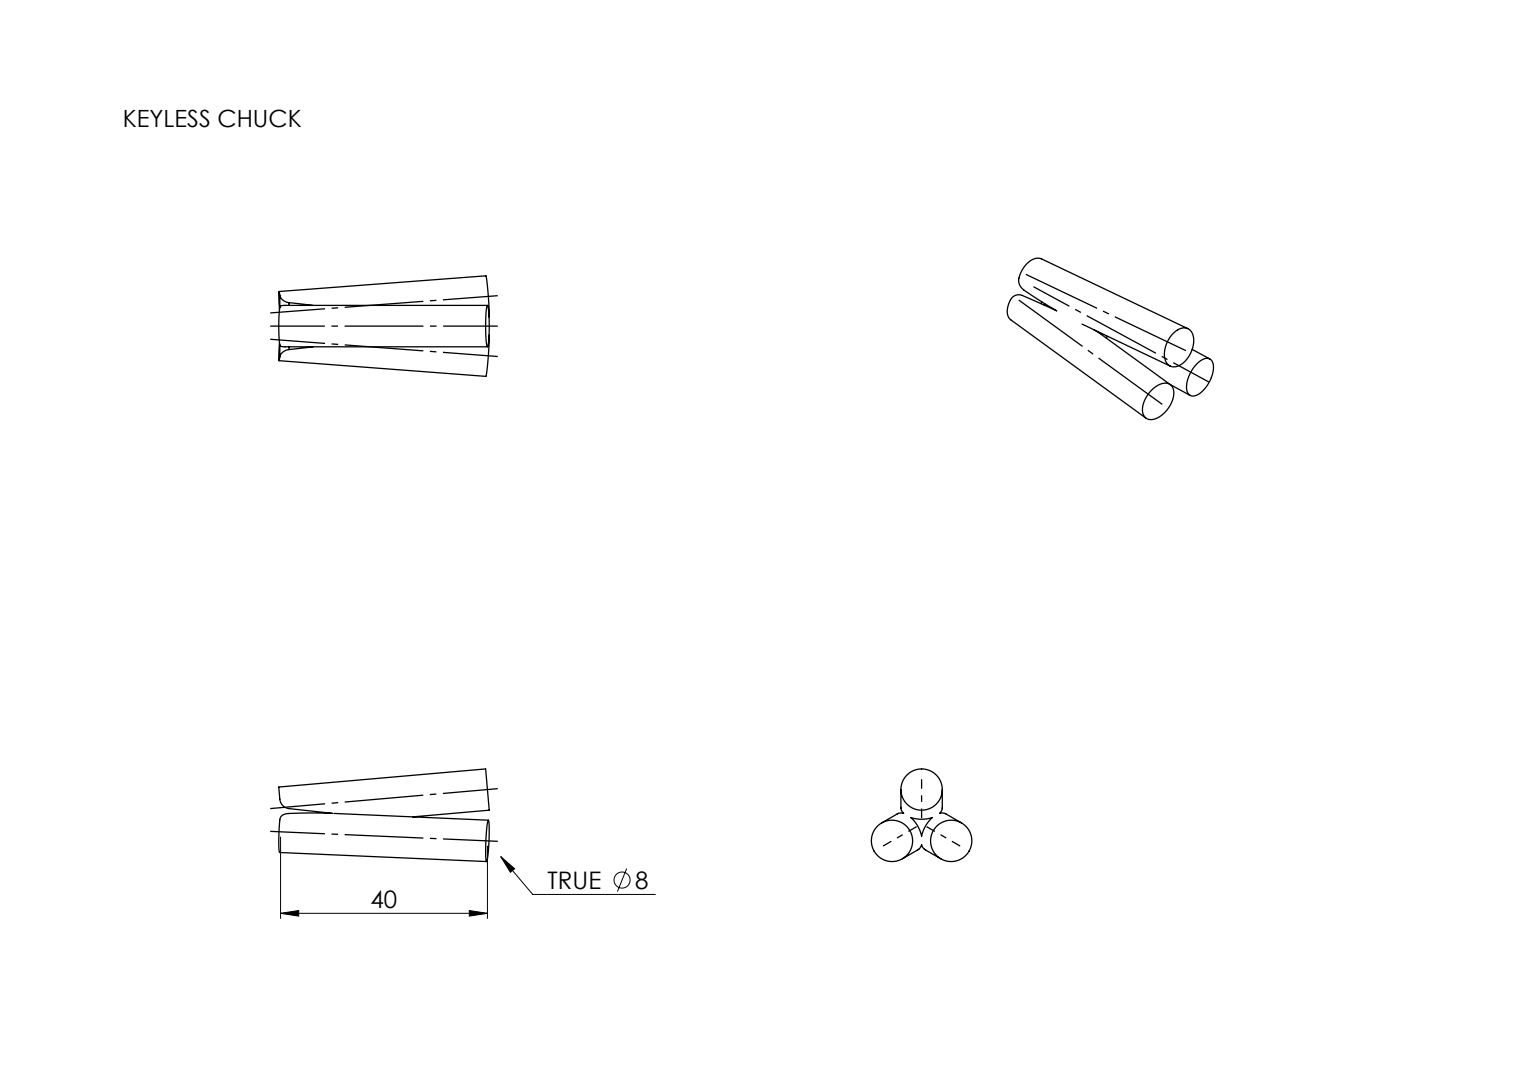
ISO-10303-21;
HEADER;
FILE_DESCRIPTION (('STEP AP214'),
    '1' );
FILE_NAME ('Keyless Chuck.step',
    '2026-10-05T20:22:16',
    ( '' ),
    ( '' ),
    'SwSTEP 2.0',
    'SolidWorks 2026',
    '' );
FILE_SCHEMA (( 'AUTOMOTIVE_DESIGN' ));
ENDSEC;

DATA;
#15=AXIS2_PLACEMENT_3D ( 'NONE', #2563, #7954, #5300 ) ;
#46=SHAPE_DEFINITION_REPRESENTATION ( #2904, #690 ) ;
#51=AXIS2_PLACEMENT_3D ( 'NONE', #14892, #2772, #6847 ) ;
#157=STYLED_ITEM ( 'NONE', ( #14231 ), #11475 ) ;
#195=DIRECTION ( 'NONE',  ( 0.1091791256177803149, 0.9940220915700701543, 0.000000000000000000 ) ) ;
#229=CARTESIAN_POINT ( 'NONE',  ( -208.1430079281944074, 172.4097984991905150, 5.932774073184737595 ) ) ;
#323=ORIENTED_EDGE ( 'NONE', *, *, #15869, .T. ) ;
#367=CARTESIAN_POINT ( 'NONE',  ( -206.3689767832464668, 174.5534660175772785, 3.987129972734268168 ) ) ;
#396=CARTESIAN_POINT ( 'NONE',  ( -206.1506185320109239, 176.5415102007174255, 53.79077198841061147 ) ) ;
#448=CARTESIAN_POINT ( 'NONE',  ( -207.5170152892447959, 175.0764231502095072, 3.989746324742934558 ) ) ;
#456=AXIS2_PLACEMENT_3D ( 'NONE', #11979, #6311, #7995 ) ;
#518=CIRCLE ( 'NONE', #8724, 4.000000000000001776 ) ;
#542=CARTESIAN_POINT ( 'NONE',  ( -187.6513770290094385, 171.1853623553244006, 0.7576236986490064718 ) ) ;
#607=EDGE_CURVE ( 'NONE', #15092, #6530, #17001, .T. ) ;
#637=CARTESIAN_POINT ( 'NONE',  ( -207.6770884633517085, 166.3723159270569738, -1.150078995496658596 ) ) ;
#638=CARTESIAN_POINT ( 'NONE',  ( -207.7508999721942189, 175.3364228813296108, 3.959069933371625716 ) ) ;
#664=CARTESIAN_POINT ( 'NONE',  ( -206.3689767832464668, 174.5534660175772785, 53.79077198841061147 ) ) ;
#686=( NAMED_UNIT ( * ) SI_UNIT ( $, .STERADIAN. ) SOLID_ANGLE_UNIT ( ) );
#690=SHAPE_REPRESENTATION ( 'Keyless Chuck', ( #3583 ), #12675 ) ;
#739=CARTESIAN_POINT ( 'NONE',  ( -195.2299705378136991, 173.3300053194287784, 3.811055608065186728 ) ) ;
#766=CARTESIAN_POINT ( 'NONE',  ( -207.6513770290094669, 172.0602489905835739, -0.7577244044828647107 ) ) ;
#773=AXIS2_PLACEMENT_3D ( 'NONE', #13462, #4256, #5749 ) ;
#777=( LENGTH_UNIT ( ) NAMED_UNIT ( * ) SI_UNIT ( .MILLI., .METRE. ) );
#789=DIRECTION ( 'NONE',  ( 0.9961946980917461003, 0.08715574274765185148, 0.000000000000000000 ) ) ;
#824=CIRCLE ( 'NONE', #2229, 3.999999999999985789 ) ;
#840=ORIENTED_EDGE ( 'NONE', *, *, #4013, .T. ) ;
#841=CARTESIAN_POINT ( 'NONE',  ( -207.2467692809710229, 174.8522807748693708, -4.001497440111938531 ) ) ;
#849=EDGE_CURVE ( 'NONE', #13616, #7959, #8196, .T. ) ;
#859=DIRECTION ( 'NONE',  ( -0.08715574274764689711, 0.9961946980917465444, 0.000000000000000000 ) ) ;
#924=ORIENTED_EDGE ( 'NONE', *, *, #4888, .T. ) ;
#935=EDGE_CURVE ( 'NONE', #15663, #15092, #15839, .T. ) ;
#944=FACE_OUTER_BOUND ( 'NONE', #7191, .T. ) ;
#1009=ORIENTED_EDGE ( 'NONE', *, *, #607, .T. ) ;
#1035=FACE_OUTER_BOUND ( 'NONE', #10686, .T. ) ;
#1091=DIRECTION ( 'NONE',  ( 0.000000000000000000, 0.8660254037844363761, 0.5000000000000039968 ) ) ;
#1110=SURFACE_STYLE_FILL_AREA ( #5093 ) ;
#1139=CARTESIAN_POINT ( 'NONE',  ( -206.6025269363104258, 173.6007587957575993, -4.555677747302790515 ) ) ;
#1184=FACE_OUTER_BOUND ( 'NONE', #5191, .T. ) ;
#1208=ORIENTED_EDGE ( 'NONE', *, *, #14941, .T. ) ;
#1212=PRESENTATION_STYLE_ASSIGNMENT (( #2453 ) ) ;
#1213=DIRECTION ( 'NONE',  ( -0.08715574274765344742, -0.4980973490458779906, 0.8627299156628184251 ) ) ;
#1262=CARTESIAN_POINT ( 'NONE',  ( -208.1430079281944074, 176.3671987152221448, 3.647967993167786194 ) ) ;
#1265=ORIENTED_EDGE ( 'NONE', *, *, #4152, .T. ) ;
#1297=STYLED_ITEM ( 'NONE', ( #15804 ), #5484 ) ;
#1302=CYLINDRICAL_SURFACE ( 'NONE', #11228, 3.999999999999999556 ) ;
#1304=CARTESIAN_POINT ( 'NONE',  ( -208.0000000000000853, 170.0678595944000620, 2.693195258168412654 ) ) ;
#1332=APPLICATION_CONTEXT ( 'automotive_design' ) ;
#1368=AXIS2_PLACEMENT_3D ( 'NONE', #14284, #2415, #6495 ) ;
#1393=AXIS2_PLACEMENT_3D ( 'NONE', #396, #7302, #5984 ) ;
#1460=VERTEX_POINT ( 'NONE', #542 ) ;
#1523=ORIENTED_EDGE ( 'NONE', *, *, #3971, .T. ) ;
#1571=FACE_OUTER_BOUND ( 'NONE', #7575, .T. ) ;
#1581=FACE_OUTER_BOUND ( 'NONE', #1905, .T. ) ;
#1616=DIRECTION ( 'NONE',  ( -0.9940220915700700433, 0.1091791256177803010, 0.000000000000000000 ) ) ;
#1619=EDGE_CURVE ( 'NONE', #10750, #7725, #11750, .T. ) ;
#1633=PRODUCT_DEFINITION_FORMATION_WITH_SPECIFIED_SOURCE ( 'ANY', '', #8716, .NOT_KNOWN. ) ;
#1648=CARTESIAN_POINT ( 'NONE',  ( -206.8260782938592968, 173.5737298318736350, 4.615523682683083884 ) ) ;
#1664=CARTESIAN_POINT ( 'NONE',  ( -208.1243352336975079, 166.1145920781434029, 2.051787360128269899 ) ) ;
#1670=AXIS2_PLACEMENT_3D ( 'NONE', #11861, #14612, #14871 ) ;
#1700=EDGE_LOOP ( 'NONE', ( #10050, #15247, #3822 ) ) ;
#1706=CARTESIAN_POINT ( 'NONE',  ( -207.9324504923922916, 166.2413418076914979, -1.515671747849433926 ) ) ;
#1748=CARTESIAN_POINT ( 'NONE',  ( -207.9328752093750836, 166.2410986792852725, 1.516464574996131409 ) ) ;
#1830=MECHANICAL_DESIGN_GEOMETRIC_PRESENTATION_REPRESENTATION('',(#15396),#8611);
#1858=ORIENTED_EDGE ( 'NONE', *, *, #13622, .T. ) ;
#1899=ADVANCED_FACE ( 'NONE', ( #1035 ), #13080, .T. ) ;
#1905=EDGE_LOOP ( 'NONE', ( #3437, #5081, #4944 ) ) ;
#1946=FACE_OUTER_BOUND ( 'NONE', #7383, .T. ) ;
#1962=CARTESIAN_POINT ( 'NONE',  ( -206.8291083847463767, 174.6458110457699320, 3.997382128395213563 ) ) ;
#2102=CARTESIAN_POINT ( 'NONE',  ( -206.3689767832464668, 173.6103877383153247, 4.531616471133065538 ) ) ;
#2132=EDGE_CURVE ( 'NONE', #16060, #12961, #14037, .T. ) ;
#2147=CLOSED_SHELL ( 'NONE', ( #14473, #16622, #2895, #16851, #8239, #12846 ) ) ;
#2222=ORIENTED_EDGE ( 'NONE', *, *, #14690, .T. ) ;
#2229=AXIS2_PLACEMENT_3D ( 'NONE', #2965, #8362, #5374 ) ;
#2260=( NAMED_UNIT ( * ) PLANE_ANGLE_UNIT ( ) SI_UNIT ( $, .RADIAN. ) );
#2263=DIRECTION ( 'NONE',  ( 0.9961946980917461003, -0.04357787137382628656, 0.07547908730516766918 ) ) ;
#2279=EDGE_LOOP ( 'NONE', ( #3266, #2377, #8282 ) ) ;
#2286=ORIENTED_EDGE ( 'NONE', *, *, #6993, .T. ) ;
#2301=ORIENTED_EDGE ( 'NONE', *, *, #5852, .T. ) ;
#2354=EDGE_CURVE ( 'NONE', #15563, #4664, #11297, .T. ) ;
#2357=CARTESIAN_POINT ( 'NONE',  ( -206.3689767832464668, 174.5534660175772785, -3.987129972734268168 ) ) ;
#2377=ORIENTED_EDGE ( 'NONE', *, *, #13820, .T. ) ;
#2389=CYLINDRICAL_SURFACE ( 'NONE', #1670, 2.000000000000001776 ) ;
#2415=DIRECTION ( 'NONE',  ( 0.1091791256177803288, -0.4970110457850271390, -0.8608483832226269117 ) ) ;
#2416=( GEOMETRIC_REPRESENTATION_CONTEXT ( 3 ) GLOBAL_UNCERTAINTY_ASSIGNED_CONTEXT ( ( #11805 ) ) GLOBAL_UNIT_ASSIGNED_CONTEXT ( ( #777, #6172, #686 ) ) REPRESENTATION_CONTEXT ( 'NONE', 'WORKASPACE' ) );
#2424=UNCERTAINTY_MEASURE_WITH_UNIT (LENGTH_MEASURE( 1.000000000000000082E-05 ), #9338, 'distance_accuracy_value', 'NONE');
#2453=SURFACE_STYLE_USAGE ( .BOTH. , #10588 ) ;
#2470=VERTEX_POINT ( 'NONE', #6364 ) ;
#2494=B_SPLINE_CURVE_WITH_KNOTS ( 'NONE', 3,
 ( #6445, #17249, #7857, #10785, #13268, #9183, #9275, #3786, #15833, #5124, #15917, #16195, #1139, #5029 ),
 .UNSPECIFIED., .F., .F.,
 ( 4, 2, 2, 2, 2, 2, 4 ),
 ( 0.000000000000000000, 0.0006954478661160458245, 0.001043171799174067707, 0.001390895732232089697, 0.001738619665290111688, 0.002086343598348133679, 0.002781791464464176359 ),
 .UNSPECIFIED. ) ;
#2514=CARTESIAN_POINT ( 'NONE',  ( -207.6770884633516516, 175.2440045654562368, -3.971992828049704993 ) ) ;
#2529=EDGE_CURVE ( 'NONE', #12961, #8416, #16124, .T. ) ;
#2558=AXIS2_PLACEMENT_3D ( 'NONE', #1304, #5022, #1213 ) ;
#2563=CARTESIAN_POINT ( 'NONE',  ( -208.0000000000000853, 123.4836845632602262, -24.20219073603711735 ) ) ;
#2589=FACE_OUTER_BOUND ( 'NONE', #7027, .T. ) ;
#2608=ORIENTED_EDGE ( 'NONE', *, *, #6258, .T. ) ;
#2655=DIRECTION ( 'NONE',  ( -0.08715574274764661955, -0.4980973490458647235, -0.8627299156628267518 ) ) ;
#2663=PRESENTATION_STYLE_ASSIGNMENT (( #7884 ) ) ;
#2666=DIRECTION ( 'NONE',  ( 0.9961946980917461003, -0.04357787137382628656, 0.07547908730516766918 ) ) ;
#2747=CARTESIAN_POINT ( 'NONE',  ( -208.0000000000000853, 174.7326106162513497, 0.000000000000000000 ) ) ;
#2751=CARTESIAN_POINT ( 'NONE',  ( -206.3689767832464668, 173.6103877383153531, -4.531616471133038004 ) ) ;
#2760=AXIS2_PLACEMENT_3D ( 'NONE', #15474, #12819, #3354 ) ;
#2772=DIRECTION ( 'NONE',  ( 0.9961946980917464334, 0.08715574274764831264, 0.000000000000000000 ) ) ;
#2796=AXIS2_PLACEMENT_3D ( 'NONE', #9390, #2666, #8056 ) ;
#2809=ORIENTED_EDGE ( 'NONE', *, *, #4152, .F. ) ;
#2813=CARTESIAN_POINT ( 'NONE',  ( -207.2426727481553996, 166.5388791023002852, 0.8050770646283873511 ) ) ;
#2859=ORIENTED_EDGE ( 'NONE', *, *, #17159, .T. ) ;
#2894=CARTESIAN_POINT ( 'NONE',  ( -207.7508999721942189, 166.3372983242019529, 1.236577052156976331 ) ) ;
#2895=ADVANCED_FACE ( 'NONE', ( #6536 ), #9267, .T. ) ;
#2904=PRODUCT_DEFINITION_SHAPE ( 'NONE', 'NONE',  #4806 ) ;
#2965=CARTESIAN_POINT ( 'NONE',  ( -168.0000000000000284, 178.2321571572880146, 0.000000000000000000 ) ) ;
#2994=DIRECTION ( 'NONE',  ( -0.08715574274764689711, 0.9961946980917465444, 0.000000000000000000 ) ) ;
#3095=DIRECTION ( 'NONE',  ( 0.9961946980917465444, -0.04357787137382451714, 0.07547908730516460218 ) ) ;
#3142=APPLICATION_CONTEXT ( 'automotive_design' ) ;
#3156=ORIENTED_EDGE ( 'NONE', *, *, #3757, .F. ) ;
#3173=EDGE_CURVE ( 'NONE', #1460, #13560, #8889, .T. ) ;
#3177=FACE_OUTER_BOUND ( 'NONE', #12170, .T. ) ;
#3266=ORIENTED_EDGE ( 'NONE', *, *, #3738, .F. ) ;
#3269=MECHANICAL_DESIGN_GEOMETRIC_PRESENTATION_REPRESENTATION('',(#157),#2416);
#3278=ORIENTED_EDGE ( 'NONE', *, *, #3173, .F. ) ;
#3350=SURFACE_STYLE_USAGE ( .BOTH. , #11477 ) ;
#3354=DIRECTION ( 'NONE',  ( -0.08715574274764828488, -0.4980973490458772135, 0.8627299156628193133 ) ) ;
#3371=CARTESIAN_POINT ( 'NONE',  ( -207.6513770290094669, 170.7478318238843542, 4.898587196589412829E-16 ) ) ;
#3404=LINE ( 'NONE', #12602, #7236 ) ;
#3437=ORIENTED_EDGE ( 'NONE', *, *, #13167, .F. ) ;
#3583=AXIS2_PLACEMENT_3D ( 'NONE', #5482, #6893, #8222 ) ;
#3595=CARTESIAN_POINT ( 'NONE',  ( -167.6513770290094385, 170.3104757200652273, -2.272971801780872880 ) ) ;
#3667=AXIS2_PLACEMENT_3D ( 'NONE', #8932, #14257, #10184 ) ;
#3693=ORIENTED_EDGE ( 'NONE', *, *, #16219, .F. ) ;
#3700=VECTOR ( 'NONE', #11958, 1000.000000000000000 ) ;
#3705=EDGE_CURVE ( 'NONE', #2470, #13560, #518, .T. ) ;
#3714=ORIENTED_EDGE ( 'NONE', *, *, #12478, .T. ) ;
#3738=EDGE_CURVE ( 'NONE', #12853, #7172, #10395, .T. ) ;
#3757=EDGE_CURVE ( 'NONE', #5890, #4664, #5665, .T. ) ;
#3783=DIRECTION ( 'NONE',  ( -0.08715574274764661955, -0.4980973490458647235, -0.8627299156628267518 ) ) ;
#3786=CARTESIAN_POINT ( 'NONE',  ( -207.5170152892447675, 173.3511749993040496, -4.985818809087040115 ) ) ;
#3822=ORIENTED_EDGE ( 'NONE', *, *, #1619, .F. ) ;
#3839=MECHANICAL_DESIGN_GEOMETRIC_PRESENTATION_REPRESENTATION('',(#1297),#13733);
#3886=CARTESIAN_POINT ( 'NONE',  ( -187.6513770290094669, 169.2829632032627103, 0.3407269638998700612 ) ) ;
#3911=VECTOR ( 'NONE', #12611, 1000.000000000000000 ) ;
#3914=( NAMED_UNIT ( * ) SI_UNIT ( $, .STERADIAN. ) SOLID_ANGLE_UNIT ( ) );
#3971=EDGE_CURVE ( 'NONE', #12127, #1460, #5551, .T. ) ;
#3978=AXIS2_PLACEMENT_3D ( 'NONE', #8826, #8563, #16727 ) ;
#4013=EDGE_CURVE ( 'NONE', #10750, #5523, #14167, .T. ) ;
#4023=CARTESIAN_POINT ( 'NONE',  ( -207.8780901672883488, 175.5271247293819386, 3.924367008119225453 ) ) ;
#4035=ORIENTED_EDGE ( 'NONE', *, *, #15780, .T. ) ;
#4127=CARTESIAN_POINT ( 'NONE',  ( -207.6770884633517653, 173.2520093125383198, 5.122071823546326286 ) ) ;
#4152=EDGE_CURVE ( 'NONE', #4664, #15793, #8244, .T. ) ;
#4193=ORIENTED_EDGE ( 'NONE', *, *, #8859, .F. ) ;
#4205=B_SPLINE_CURVE_WITH_KNOTS ( 'NONE', 3,
 ( #8099, #12190, #1648, #10846, #16259, #4127, #9427, #13517, #9512, #8194, #15086, #229 ),
 .UNSPECIFIED., .F., .F.,
 ( 4, 2, 2, 2, 2, 4 ),
 ( 0.000000000000000000, 0.0006954760458706750904, 0.001390952091741350181, 0.001738690114676716024, 0.002086428137612082300, 0.002781904183482815287 ),
 .UNSPECIFIED. ) ;
#4256=DIRECTION ( 'NONE',  ( 0.000000000000000000, 0.8660254037844363761, 0.5000000000000041078 ) ) ;
#4290=ORIENTED_EDGE ( 'NONE', *, *, #2132, .F. ) ;
#4328=DIRECTION ( 'NONE',  ( -0.08715574274764828488, -0.4980973490458772135, 0.8627299156628193133 ) ) ;
#4397=DIRECTION ( 'NONE',  ( -0.08715574274765354457, -0.4980973490458646125, -0.8627299156628260857 ) ) ;
#4408=CARTESIAN_POINT ( 'NONE',  ( -206.8291083847463199, 166.6494249078165808, 0.6193335608963369543 ) ) ;
#4417=( BOUNDED_CURVE ( )  B_SPLINE_CURVE ( 3, ( #9196, #6639, #739, #9379 ),
 .UNSPECIFIED., .F., .F. ) 
 B_SPLINE_CURVE_WITH_KNOTS ( ( 4, 4 ),
 ( 0.000000000000000000, 1.490556265852237994 ),
 .UNSPECIFIED. ) 
 CURVE ( )  GEOMETRIC_REPRESENTATION_ITEM ( )  RATIONAL_B_SPLINE_CURVE ( ( 1.000000000000000000, 0.8232662051119113977, 0.8232662051119113977, 1.000000000000000000 ) ) 
 REPRESENTATION_ITEM ( '' )  );
#4445=ORIENTED_EDGE ( 'NONE', *, *, #17458, .F. ) ;
#4448=CARTESIAN_POINT ( 'NONE',  ( -206.3689767832464668, 166.7044760491588704, -0.5444864983988328966 ) ) ;
#4449=DIRECTION ( 'NONE',  ( -0.08715574274765354457, -0.4980973490458646125, -0.8627299156628260857 ) ) ;
#4469=ORIENTED_EDGE ( 'NONE', *, *, #15780, .F. ) ;
#4496=CARTESIAN_POINT ( 'NONE',  ( -207.5170152892447675, 166.4407316555380589, 0.9960724843441398635 ) ) ;
#4557=ORIENTED_EDGE ( 'NONE', *, *, #13622, .F. ) ;
#4624=CARTESIAN_POINT ( 'NONE',  ( -207.4300157105866447, 174.9998640698394468, 3.994873866052218947 ) ) ;
#4635=CARTESIAN_POINT ( 'NONE',  ( -207.6513770290094669, 172.0602489905835171, 0.7577244044828906899 ) ) ;
#4664=VERTEX_POINT ( 'NONE', #11365 ) ;
#4806=PRODUCT_DEFINITION ( 'UNKNOWN', '', #1633, #16115 ) ;
#4847=DIRECTION ( 'NONE',  ( 0.9961946980917465444, -0.04357787137382451714, 0.07547908730516460218 ) ) ;
#4852=CARTESIAN_POINT ( 'NONE',  ( -187.6513770290094669, 172.4976050944027008, -2.196701325097758062 ) ) ;
#4888=EDGE_CURVE ( 'NONE', #7725, #17193, #10115, .T. ) ;
#4896=ADVANCED_FACE ( 'NONE', ( #5768 ), #15411, .T. ) ;
#4898=LINE ( 'NONE', #11887, #8985 ) ;
#4944=ORIENTED_EDGE ( 'NONE', *, *, #2354, .F. ) ;
#4975=ORIENTED_EDGE ( 'NONE', *, *, #13167, .T. ) ;
#5022=DIRECTION ( 'NONE',  ( 0.9961946980917461003, -0.04357787137382628656, 0.07547908730516766918 ) ) ;
#5029=CARTESIAN_POINT ( 'NONE',  ( -206.3689767832464668, 173.6103877383153531, -4.531616471133038004 ) ) ;
#5039=ORIENTED_EDGE ( 'NONE', *, *, #10242, .F. ) ;
#5081=ORIENTED_EDGE ( 'NONE', *, *, #3757, .T. ) ;
#5093=FILL_AREA_STYLE ('',( #5264 ) ) ;
#5124=CARTESIAN_POINT ( 'NONE',  ( -207.2426727481553996, 173.4675081614032877, -4.805322917016542128 ) ) ;
#5191=EDGE_LOOP ( 'NONE', ( #9064, #9073, #1208, #3714, #840, #4469 ) ) ;
#5264=FILL_AREA_STYLE_COLOUR ( '', #16842 ) ;
#5282=STYLED_ITEM ( 'NONE', ( #1212 ), #12908 ) ;
#5300=DIRECTION ( 'NONE',  ( -0.9940220915700700433, -0.05458956280889060153, 0.09455189634796991316 ) ) ;
#5306=AXIS2_PLACEMENT_3D ( 'NONE', #9251, #4847, #8988 ) ;
#5319=CARTESIAN_POINT ( 'NONE',  ( -167.6513770290094385, 174.2473783649210759, 4.898587196589412829E-16 ) ) ;
#5374=DIRECTION ( 'NONE',  ( -0.08715574274764689711, 0.9961946980917465444, 0.000000000000000000 ) ) ;
#5430=DIRECTION ( 'NONE',  ( -0.000000000000000000, -0.000000000000000000, 1.000000000000000000 ) ) ;
#5433=CARTESIAN_POINT ( 'NONE',  ( -208.3486229709906468, 168.0754701982166068, -6.144114920819718328 ) ) ;
#5482=CARTESIAN_POINT ( 'NONE',  ( 0.000000000000000000, 0.000000000000000000, 0.000000000000000000 ) ) ;
#5484=MANIFOLD_SOLID_BREP ( 'CirPattern1[2]', #16287 ) ;
#5493=CIRCLE ( 'NONE', #8308, 3.999999999999998668 ) ;
#5523=VERTEX_POINT ( 'NONE', #17393 ) ;
#5524=VECTOR ( 'NONE', #2263, 1000.000000000000000 ) ;
#5543=ORIENTED_EDGE ( 'NONE', *, *, #14941, .F. ) ;
#5551=( BOUNDED_CURVE ( )  B_SPLINE_CURVE ( 3, ( #2102, #9980, #10324, #6181 ),
 .UNSPECIFIED., .F., .F. ) 
 B_SPLINE_CURVE_WITH_KNOTS ( ( 4, 4 ),
 ( 4.792629041327348460, 6.283185307179586232 ),
 .UNSPECIFIED. ) 
 CURVE ( )  GEOMETRIC_REPRESENTATION_ITEM ( )  RATIONAL_B_SPLINE_CURVE ( ( 1.000000000000000000, 0.8232662051119113977, 0.8232662051119113977, 1.000000000000000000 ) ) 
 REPRESENTATION_ITEM ( '' )  );
#5555=CARTESIAN_POINT ( 'NONE',  ( -208.0711340499744608, 166.1567726281969613, 1.827846230796970950 ) ) ;
#5581=PLANE ( 'NONE',  #5807 ) ;
#5602=MECHANICAL_DESIGN_GEOMETRIC_PRESENTATION_REPRESENTATION('',(#5282),#8948);
#5665=LINE ( 'NONE', #10871, #15778 ) ;
#5743=DIRECTION ( 'NONE',  ( 0.9961946980917465444, 0.08715574274764831264, 0.000000000000000000 ) ) ;
#5749=DIRECTION ( 'NONE',  ( -1.000000000000000000, 0.000000000000000000, 0.000000000000000000 ) ) ;
#5768=FACE_OUTER_BOUND ( 'NONE', #9574, .T. ) ;
#5783=ORIENTED_EDGE ( 'NONE', *, *, #8859, .T. ) ;
#5807=AXIS2_PLACEMENT_3D ( 'NONE', #8307, #8579, #13991 ) ;
#5811=CARTESIAN_POINT ( 'NONE',  ( -208.1430079281944074, 166.0913325906388422, 2.284806080016937635 ) ) ;
#5852=EDGE_CURVE ( 'NONE', #7172, #7959, #3404, .T. ) ;
#5857=CARTESIAN_POINT ( 'NONE',  ( -207.2426727481553428, 174.8619425413479860, 4.000245852388181866 ) ) ;
#5887=LINE ( 'NONE', #7393, #3911 ) ;
#5890=VERTEX_POINT ( 'NONE', #13045 ) ;
#5960=CARTESIAN_POINT ( 'NONE',  ( -208.3486229709906468, 178.7173894086183168, 0.000000000000000000 ) ) ;
#5984=DIRECTION ( 'NONE',  ( -1.000000000000000000, 0.000000000000000000, 0.000000000000000000 ) ) ;
#6054=FACE_OUTER_BOUND ( 'NONE', #11289, .T. ) ;
#6100=EDGE_CURVE ( 'NONE', #12567, #7725, #6916, .T. ) ;
#6162=DIRECTION ( 'NONE',  ( 0.9961946980917461003, -0.04357787137382628656, 0.07547908730516766918 ) ) ;
#6172=( NAMED_UNIT ( * ) PLANE_ANGLE_UNIT ( ) SI_UNIT ( $, .RADIAN. ) );
#6181=CARTESIAN_POINT ( 'NONE',  ( -187.6513770290094385, 171.1853623553244006, 0.7576236986490064718 ) ) ;
#6182=DIRECTION ( 'NONE',  ( -0.08715574274764831264, -0.4980973490458652231, -0.8627299156628261967 ) ) ;
#6247=( NAMED_UNIT ( * ) SI_UNIT ( $, .STERADIAN. ) SOLID_ANGLE_UNIT ( ) );
#6258=EDGE_CURVE ( 'NONE', #8416, #12853, #17430, .T. ) ;
#6311=DIRECTION ( 'NONE',  ( 0.9961946980917461003, 0.08715574274765185148, 0.000000000000000000 ) ) ;
#6324=CARTESIAN_POINT ( 'NONE',  ( -208.0000000000000853, 170.0678595944000620, -2.693195258168412654 ) ) ;
#6333=DIRECTION ( 'NONE',  ( 0.9961946980917461003, 0.08715574274765185148, 0.000000000000000000 ) ) ;
#6347=CARTESIAN_POINT ( 'NONE',  ( -168.0000000000000284, 168.3180863238818006, -5.723891464432168341 ) ) ;
#6353=AXIS2_PLACEMENT_3D ( 'NONE', #14008, #12583, #4449 ) ;
#6364=CARTESIAN_POINT ( 'NONE',  ( -168.3486229709906183, 166.3256969276982034, 9.174811127083433604 ) ) ;
#6424=CIRCLE ( 'NONE', #5306, 4.000000000000001776 ) ;
#6445=CARTESIAN_POINT ( 'NONE',  ( -208.1430079281944074, 172.4097984991905435, -5.932774073184737595 ) ) ;
#6495=DIRECTION ( 'NONE',  ( -0.9940220915700700433, -0.05458956280888926926, -0.09455189634797064868 ) ) ;
#6530=VERTEX_POINT ( 'NONE', #5319 ) ;
#6535=FILL_AREA_STYLE ('',( #7849 ) ) ;
#6536=FACE_OUTER_BOUND ( 'NONE', #8429, .T. ) ;
#6589=CYLINDRICAL_SURFACE ( 'NONE', #456, 3.999999999999988010 ) ;
#6616=DIRECTION ( 'NONE',  ( -0.08715574274764831264, 0.9961946980917464334, 0.000000000000000000 ) ) ;
#6618=( LENGTH_UNIT ( ) NAMED_UNIT ( * ) SI_UNIT ( .MILLI., .METRE. ) );
#6639=CARTESIAN_POINT ( 'NONE',  ( -187.6513770290094669, 172.4976050944027008, 2.196701325097758950 ) ) ;
#6658=VERTEX_POINT ( 'NONE', #15387 ) ;
#6664=CIRCLE ( 'NONE', #14021, 3.999999999999985789 ) ;
#6738=FACE_OUTER_BOUND ( 'NONE', #13787, .T. ) ;
#6807=EDGE_CURVE ( 'NONE', #7959, #13616, #5493, .T. ) ;
#6847=DIRECTION ( 'NONE',  ( -0.08715574274764831264, 0.9961946980917464334, 0.000000000000000000 ) ) ;
#6888=ADVANCED_FACE ( 'NONE', ( #10325 ), #14498, .F. ) ;
#6893=DIRECTION ( 'NONE',  ( 0.000000000000000000, 0.000000000000000000, 1.000000000000000000 ) ) ;
#6901=AXIS2_PLACEMENT_3D ( 'NONE', #7758, #11835, #6182 ) ;
#6916=LINE ( 'NONE', #14727, #15721 ) ;
#6993=EDGE_CURVE ( 'NONE', #8416, #16060, #8704, .T. ) ;
#7027=EDGE_LOOP ( 'NONE', ( #15745, #16522, #9145, #10788, #11004, #1265 ) ) ;
#7101=CARTESIAN_POINT ( 'NONE',  ( -207.6775903968322154, 175.2446381608502008, 3.971903508328557653 ) ) ;
#7113=CARTESIAN_POINT ( 'NONE',  ( -187.6513770290094669, 171.1853623553243722, -0.7576236986489900405 ) ) ;
#7138=CARTESIAN_POINT ( 'NONE',  ( -206.3689767832464668, 166.7044760491588988, 0.5444864983987496299 ) ) ;
#7172=VERTEX_POINT ( 'NONE', #5433 ) ;
#7182=FACE_OUTER_BOUND ( 'NONE', #17093, .T. ) ;
#7191=EDGE_LOOP ( 'NONE', ( #4445, #1009, #7621, #7416, #17238, #924 ) ) ;
#7236=VECTOR ( 'NONE', #13865, 1000.000000000000000 ) ;
#7284=LINE ( 'NONE', #4635, #9162 ) ;
#7302=DIRECTION ( 'NONE',  ( 0.000000000000000000, 0.000000000000000000, -1.000000000000000000 ) ) ;
#7344=ORIENTED_EDGE ( 'NONE', *, *, #2529, .T. ) ;
#7383=EDGE_LOOP ( 'NONE', ( #9937, #12708 ) ) ;
#7393=CARTESIAN_POINT ( 'NONE',  ( -208.1430079281944074, 169.2505655449146786, -4.108790076600865149 ) ) ;
#7416=ORIENTED_EDGE ( 'NONE', *, *, #4013, .F. ) ;
#7551=CYLINDRICAL_SURFACE ( 'NONE', #773, 2.000000000000001776 ) ;
#7557=CARTESIAN_POINT ( 'NONE',  ( -206.8260782938593820, 174.6444607475611406, -3.997336900281264427 ) ) ;
#7575=EDGE_LOOP ( 'NONE', ( #1523, #2859, #16822 ) ) ;
#7621=ORIENTED_EDGE ( 'NONE', *, *, #14742, .F. ) ;
#7725=VERTEX_POINT ( 'NONE', #14708 ) ;
#7748=CARTESIAN_POINT ( 'NONE',  ( -195.2299705378136991, 173.3300053194287784, -3.811055608065186728 ) ) ;
#7758=CARTESIAN_POINT ( 'NONE',  ( -208.0000000000000853, 170.0678595944000620, -2.693195258168412654 ) ) ;
#7779=COLOUR_RGB ( '', 0.31764706, 0.68627451, 0.89019608) ;
#7849=FILL_AREA_STYLE_COLOUR ( '', #8146 ) ;
#7857=CARTESIAN_POINT ( 'NONE',  ( -208.0711340499744040, 172.7728173183454601, -5.647621413624758446 ) ) ;
#7861=VECTOR ( 'NONE', #789, 1000.000000000000000 ) ;
#7884=SURFACE_STYLE_USAGE ( .BOTH. , #16216 ) ;
#7904=PLANE ( 'NONE',  #51 ) ;
#7912=CARTESIAN_POINT ( 'NONE',  ( -206.3689767832464668, 173.6103877383153247, 4.531616471133065538 ) ) ;
#7954=DIRECTION ( 'NONE',  ( 0.1091791256177803426, -0.4970110457850390184, 0.8608483832226199173 ) ) ;
#7959=VERTEX_POINT ( 'NONE', #17071 ) ;
#7995=DIRECTION ( 'NONE',  ( -0.08715574274765379437, 0.9961946980917459893, 0.000000000000000000 ) ) ;
#8000=ORIENTED_EDGE ( 'NONE', *, *, #3705, .T. ) ;
#8056=DIRECTION ( 'NONE',  ( -0.08715574274765344742, -0.4980973490458779906, 0.8627299156628184251 ) ) ;
#8068=AXIS2_PLACEMENT_3D ( 'NONE', #6324, #11719, #17129 ) ;
#8078=CARTESIAN_POINT ( 'NONE',  ( -208.1243153690002714, 176.1535417859606980, -3.744436563795452866 ) ) ;
#8099=CARTESIAN_POINT ( 'NONE',  ( -206.3689767832464668, 173.6103877383153247, 4.531616471133065538 ) ) ;
#8113=CARTESIAN_POINT ( 'NONE',  ( -207.8780901672884056, 166.2720010150300425, 1.419081159745146259 ) ) ;
#8132=CARTESIAN_POINT ( 'NONE',  ( -208.0000000000000853, 174.7326106162513497, 0.000000000000000000 ) ) ;
#8146=COLOUR_RGB ( '', 0.40784314, 0.44705882, 0.49803922) ;
#8194=CARTESIAN_POINT ( 'NONE',  ( -208.0706889292728761, 172.7738155144439531, 5.646695128860279134 ) ) ;
#8196=CIRCLE ( 'NONE', #3978, 3.999999999999998668 ) ;
#8219=DIRECTION ( 'NONE',  ( 0.9961946980917464334, -0.04357787137382450326, 0.07547908730516456055 ) ) ;
#8222=DIRECTION ( 'NONE',  ( 1.000000000000000000, 0.000000000000000000, 0.000000000000000000 ) ) ;
#8239=ADVANCED_FACE ( 'NONE', ( #1571 ), #13358, .F. ) ;
#8244=B_SPLINE_CURVE_WITH_KNOTS ( 'NONE', 3,
 ( #5811, #1664, #5555, #1748, #8113, #2894, #12201, #4496, #10945, #2813, #11205, #4408, #16367, #15100 ),
 .UNSPECIFIED., .F., .F.,
 ( 4, 2, 2, 2, 2, 2, 4 ),
 ( 0.000000000000000000, 0.0006954478661160149247, 0.001043171799174032579, 0.001390895732232050232, 0.001738619665290067886, 0.002086343598348085540, 0.002781791464464176359 ),
 .UNSPECIFIED. ) ;
#8281=CARTESIAN_POINT ( 'NONE',  ( -208.0000000000000853, 170.0678595944000620, -2.693195258168412654 ) ) ;
#8282=ORIENTED_EDGE ( 'NONE', *, *, #15869, .F. ) ;
#8307=CARTESIAN_POINT ( 'NONE',  ( -168.0000000000000284, 168.3180863238818006, -5.723891464432168341 ) ) ;
#8308=AXIS2_PLACEMENT_3D ( 'NONE', #6347, #8912, #3783 ) ;
#8362=DIRECTION ( 'NONE',  ( 0.9961946980917465444, 0.08715574274764831264, 0.000000000000000000 ) ) ;
#8370=ORIENTED_EDGE ( 'NONE', *, *, #16219, .T. ) ;
#8416=VERTEX_POINT ( 'NONE', #8990 ) ;
#8429=EDGE_LOOP ( 'NONE', ( #3278, #14235, #2222, #4975, #13828, #4557 ) ) ;
#8563=DIRECTION ( 'NONE',  ( 0.9961946980917463224, -0.04357787137382344855, -0.07547908730516518505 ) ) ;
#8579=DIRECTION ( 'NONE',  ( 0.9961946980917464334, -0.04357787137382345549, -0.07547908730516519893 ) ) ;
#8611=( GEOMETRIC_REPRESENTATION_CONTEXT ( 3 ) GLOBAL_UNCERTAINTY_ASSIGNED_CONTEXT ( ( #14650 ) ) GLOBAL_UNIT_ASSIGNED_CONTEXT ( ( #12300, #14873, #3914 ) ) REPRESENTATION_CONTEXT ( 'NONE', 'WORKASPACE' ) );
#8622=ORIENTED_EDGE ( 'NONE', *, *, #5852, .F. ) ;
#8627=FACE_OUTER_BOUND ( 'NONE', #16322, .T. ) ;
#8636=CARTESIAN_POINT ( 'NONE',  ( -187.6513770290094953, 169.2829632032627956, -0.3407269638998823291 ) ) ;
#8651=B_SPLINE_CURVE_WITH_KNOTS ( 'NONE', 3,
 ( #10476, #10554, #7557, #841, #14642, #2514, #13319, #11544, #12966, #13400, #8078, #16330 ),
 .UNSPECIFIED., .F., .F.,
 ( 4, 2, 2, 2, 2, 4 ),
 ( 0.000000000000000000, 0.0006954760458707579234, 0.001390952091741515847, 0.001738690114676866294, 0.002086428137612216741, 0.002781904183482844344 ),
 .UNSPECIFIED. ) ;
#8654=CYLINDRICAL_SURFACE ( 'NONE', #9772, 3.999999999999988010 ) ;
#8691=CARTESIAN_POINT ( 'NONE',  ( -206.6025269363104826, 174.5791181652666353, 3.990821701952568468 ) ) ;
#8703=DIRECTION ( 'NONE',  ( 0.9961946980917461003, -0.04357787137382522491, -0.07547908730516825204 ) ) ;
#8704=( BOUNDED_CURVE ( )  B_SPLINE_CURVE ( 3, ( #9180, #17331, #3886, #14679 ),
 .UNSPECIFIED., .F., .F. ) 
 B_SPLINE_CURVE_WITH_KNOTS ( ( 4, 4 ),
 ( 4.792629041327348460, 6.283185307179586232 ),
 .UNSPECIFIED. ) 
 CURVE ( )  GEOMETRIC_REPRESENTATION_ITEM ( )  RATIONAL_B_SPLINE_CURVE ( ( 1.000000000000000000, 0.8232662051119113977, 0.8232662051119113977, 1.000000000000000000 ) ) 
 REPRESENTATION_ITEM ( '' )  );
#8716=PRODUCT ( 'Keyless Chuck', 'Keyless Chuck', '', ( #16340 ) ) ;
#8724=AXIS2_PLACEMENT_3D ( 'NONE', #16126, #9113, #10799 ) ;
#8826=CARTESIAN_POINT ( 'NONE',  ( -168.0000000000000284, 168.3180863238818006, -5.723891464432168341 ) ) ;
#8859=EDGE_CURVE ( 'NONE', #17193, #15663, #14211, .T. ) ;
#8889=LINE ( 'NONE', #766, #9620 ) ;
#8901=CARTESIAN_POINT ( 'NONE',  ( -208.0000000000000853, 174.7326106162513497, 0.000000000000000000 ) ) ;
#8912=DIRECTION ( 'NONE',  ( 0.9961946980917463224, -0.04357787137382344855, -0.07547908730516518505 ) ) ;
#8932=CARTESIAN_POINT ( 'NONE',  ( -208.0000000000000853, 170.0678595944000620, 2.693195258168412654 ) ) ;
#8948=( GEOMETRIC_REPRESENTATION_CONTEXT ( 3 ) GLOBAL_UNCERTAINTY_ASSIGNED_CONTEXT ( ( #12840 ) ) GLOBAL_UNIT_ASSIGNED_CONTEXT ( ( #15910, #14764, #15729 ) ) REPRESENTATION_CONTEXT ( 'NONE', 'WORKASPACE' ) );
#8985=VECTOR ( 'NONE', #1091, 999.9999999999998863 ) ;
#8988=DIRECTION ( 'NONE',  ( -0.08715574274764655016, -0.4980973490458782127, 0.8627299156628190913 ) ) ;
#8990=CARTESIAN_POINT ( 'NONE',  ( -206.3689767832464668, 166.7044760491588704, -0.5444864983988328966 ) ) ;
#9004=CARTESIAN_POINT ( 'NONE',  ( -208.3486229709906752, 178.7173894086183168, 0.000000000000000000 ) ) ;
#9064=ORIENTED_EDGE ( 'NONE', *, *, #607, .F. ) ;
#9073=ORIENTED_EDGE ( 'NONE', *, *, #935, .F. ) ;
#9113=DIRECTION ( 'NONE',  ( 0.9961946980917465444, -0.04357787137382451714, 0.07547908730516460218 ) ) ;
#9136=FACE_OUTER_BOUND ( 'NONE', #9765, .T. ) ;
#9145=ORIENTED_EDGE ( 'NONE', *, *, #3705, .F. ) ;
#9162=VECTOR ( 'NONE', #8703, 1000.000000000000000 ) ;
#9180=CARTESIAN_POINT ( 'NONE',  ( -206.3689767832464668, 166.7044760491588704, -0.5444864983988328966 ) ) ;
#9183=CARTESIAN_POINT ( 'NONE',  ( -207.7508999721942757, 173.1946085995199667, -5.195646985528586725 ) ) ;
#9196=CARTESIAN_POINT ( 'NONE',  ( -187.6513770290095238, 172.4976050944027008, 4.898587196589412829E-16 ) ) ;
#9226=FACE_OUTER_BOUND ( 'NONE', #1700, .T. ) ;
#9251=CARTESIAN_POINT ( 'NONE',  ( -168.0000000000000284, 168.3180863238817437, 5.723891464432140808 ) ) ;
#9267=CYLINDRICAL_SURFACE ( 'NONE', #2558, 4.000000000000003553 ) ;
#9275=CARTESIAN_POINT ( 'NONE',  ( -207.6775903968322439, 173.2516151616937350, -5.122575873392639423 ) ) ;
#9306=ORIENTED_EDGE ( 'NONE', *, *, #4888, .F. ) ;
#9338=( LENGTH_UNIT ( ) NAMED_UNIT ( * ) SI_UNIT ( .MILLI., .METRE. ) );
#9379=CARTESIAN_POINT ( 'NONE',  ( -206.3689767832464668, 174.5534660175772785, 3.987129972734268168 ) ) ;
#9390=CARTESIAN_POINT ( 'NONE',  ( -208.0000000000000853, 170.0678595944000620, 2.693195258168412654 ) ) ;
#9427=CARTESIAN_POINT ( 'NONE',  ( -207.7491074081026170, 173.1961128903347173, 5.193772935353458742 ) ) ;
#9432=ORIENTED_EDGE ( 'NONE', *, *, #13820, .F. ) ;
#9512=CARTESIAN_POINT ( 'NONE',  ( -207.9324504923922632, 173.0008837612440402, 5.418295114331532325 ) ) ;
#9556=FILL_AREA_STYLE_COLOUR ( '', #10293 ) ;
#9574=EDGE_LOOP ( 'NONE', ( #3693, #16958, #2608, #15967, #2301, #15440 ) ) ;
#9586=ADVANCED_FACE ( 'NONE', ( #9226 ), #7904, .F. ) ;
#9590=CARTESIAN_POINT ( 'NONE',  ( -187.6513770290094385, 173.0877615073859772, -1.855974361197849420 ) ) ;
#9613=FACE_OUTER_BOUND ( 'NONE', #15821, .T. ) ;
#9620=VECTOR ( 'NONE', #6162, 1000.000000000000000 ) ;
#9650=ADVANCED_FACE ( 'NONE', ( #7182 ), #11348, .F. ) ;
#9702=CARTESIAN_POINT ( 'NONE',  ( -206.3689767832464668, 174.5534660175772785, -3.987129972734268168 ) ) ;
#9752=ADVANCED_FACE ( 'NONE', ( #6738 ), #2389, .T. ) ;
#9765=EDGE_LOOP ( 'NONE', ( #2286, #16203, #7344 ) ) ;
#9772=AXIS2_PLACEMENT_3D ( 'NONE', #8901, #6333, #11726 ) ;
#9937=ORIENTED_EDGE ( 'NONE', *, *, #6807, .T. ) ;
#9980=CARTESIAN_POINT ( 'NONE',  ( -195.2299705378136991, 174.0696332146309260, 3.384031243670088784 ) ) ;
#10050=ORIENTED_EDGE ( 'NONE', *, *, #12478, .F. ) ;
#10085=DIRECTION ( 'NONE',  ( 0.9961946980917461003, 0.08715574274765185148, 0.000000000000000000 ) ) ;
#10115=B_SPLINE_CURVE_WITH_KNOTS ( 'NONE', 3,
 ( #1262, #12062, #17471, #16151, #4023, #638, #7101, #448, #4624, #5857, #11513, #1962, #8691, #367 ),
 .UNSPECIFIED., .F., .F.,
 ( 4, 2, 2, 2, 2, 2, 4 ),
 ( 0.000000000000000000, 0.0006954478661159615820, 0.001043171799173978802, 0.001390895732231996239, 0.001738619665290013242, 0.002086343598348030463, 0.002781791464464176359 ),
 .UNSPECIFIED. ) ;
#10184=DIRECTION ( 'NONE',  ( -0.08715574274764653628, -0.4980973490458781017, 0.8627299156628190913 ) ) ;
#10242=EDGE_CURVE ( 'NONE', #6658, #12961, #2494, .T. ) ;
#10293=COLOUR_RGB ( '', 0.40784314, 0.44705882, 0.49803922) ;
#10321=( NAMED_UNIT ( * ) SI_UNIT ( $, .STERADIAN. ) SOLID_ANGLE_UNIT ( ) );
#10324=CARTESIAN_POINT ( 'NONE',  ( -187.6513770290094669, 173.0877615073859772, 1.855974361197893607 ) ) ;
#10325=FACE_OUTER_BOUND ( 'NONE', #2279, .T. ) ;
#10359=CIRCLE ( 'NONE', #14051, 3.999999999999985789 ) ;
#10393=CARTESIAN_POINT ( 'NONE',  ( -206.3689767832464668, 166.7044760491588988, 0.5444864983987496299 ) ) ;
#10395=CIRCLE ( 'NONE', #11251, 3.999999999999998668 ) ;
#10476=CARTESIAN_POINT ( 'NONE',  ( -206.3689767832464668, 174.5534660175772785, -3.987129972734268168 ) ) ;
#10505=( NAMED_UNIT ( * ) PLANE_ANGLE_UNIT ( ) SI_UNIT ( $, .RADIAN. ) );
#10554=CARTESIAN_POINT ( 'NONE',  ( -206.6026792233873550, 174.5791348918262997, -3.990824109155664878 ) ) ;
#10588=SURFACE_SIDE_STYLE ('',( #17239 ) ) ;
#10664=SURFACE_SIDE_STYLE ('',( #1110 ) ) ;
#10686=EDGE_LOOP ( 'NONE', ( #14775, #4035 ) ) ;
#10687=SHAPE_REPRESENTATION_RELATIONSHIP ( 'NONE' , 'NONE' ,  #690, #12908 ) ;
#10707=CARTESIAN_POINT ( 'NONE',  ( -206.3689767832464668, 216.7416069248773169, -29.43343747897081286 ) ) ;
#10750=VERTEX_POINT ( 'NONE', #5960 ) ;
#10785=CARTESIAN_POINT ( 'NONE',  ( -207.9328752093750836, 173.0003187169972989, -5.418902083281068371 ) ) ;
#10788=ORIENTED_EDGE ( 'NONE', *, *, #15816, .F. ) ;
#10799=DIRECTION ( 'NONE',  ( -0.08715574274764655016, -0.4980973490458782127, 0.8627299156628190913 ) ) ;
#10846=CARTESIAN_POINT ( 'NONE',  ( -207.2467692809709376, 173.4734229514064339, 4.797581375662468339 ) ) ;
#10871=CARTESIAN_POINT ( 'NONE',  ( -208.1430079281944074, 169.2505655449146786, 4.108790076600837615 ) ) ;
#10945=CARTESIAN_POINT ( 'NONE',  ( -207.4300157105867015, 166.4745706146902364, 0.9272066051987427615 ) ) ;
#11004=ORIENTED_EDGE ( 'NONE', *, *, #2354, .T. ) ;
#11096=MANIFOLD_SOLID_BREP ( 'Fillet1', #12049 ) ;
#11128=CARTESIAN_POINT ( 'NONE',  ( -208.0000000000000853, 170.0678595944000620, 2.693195258168412654 ) ) ;
#11168=ADVANCED_FACE ( 'NONE', ( #1946 ), #5581, .T. ) ;
#11205=CARTESIAN_POINT ( 'NONE',  ( -207.1416055535977137, 166.5694718092265418, 0.7516812309923592839 ) ) ;
#11228=AXIS2_PLACEMENT_3D ( 'NONE', #8281, #16185, #4397 ) ;
#11251=AXIS2_PLACEMENT_3D ( 'NONE', #14516, #17443, #2655 ) ;
#11252=CARTESIAN_POINT ( 'NONE',  ( -206.6026792233874403, 166.6884423960484014, -0.5648693273743904397 ) ) ;
#11289=EDGE_LOOP ( 'NONE', ( #2809, #3156, #16929, #17202 ) ) ;
#11297=CIRCLE ( 'NONE', #3667, 4.000000000000002665 ) ;
#11348=PLANE ( 'NONE',  #14463 ) ;
#11365=CARTESIAN_POINT ( 'NONE',  ( -208.1430079281944074, 166.0913325906388422, 2.284806080016937635 ) ) ;
#11394=SURFACE_STYLE_FILL_AREA ( #15470 ) ;
#11418=UNCERTAINTY_MEASURE_WITH_UNIT (LENGTH_MEASURE( 1.000000000000000082E-05 ), #6618, 'distance_accuracy_value', 'NONE');
#11458=AXIS2_PLACEMENT_3D ( 'NONE', #8132, #5743, #2994 ) ;
#11475=MANIFOLD_SOLID_BREP ( 'CirPattern1[1]', #2147 ) ;
#11477=SURFACE_SIDE_STYLE ('',( #11394 ) ) ;
#11485=ORIENTED_EDGE ( 'NONE', *, *, #6100, .F. ) ;
#11513=CARTESIAN_POINT ( 'NONE',  ( -207.1416055535977989, 174.8004040394998526, 4.000449707837476332 ) ) ;
#11544=CARTESIAN_POINT ( 'NONE',  ( -207.8765633999775275, 175.5245310743884488, -3.924903759054537478 ) ) ;
#11551=ADVANCED_FACE ( 'NONE', ( #944 ), #8654, .T. ) ;
#11639=( BOUNDED_CURVE ( )  B_SPLINE_CURVE ( 3, ( #16966, #8636, #15189, #7138 ),
 .UNSPECIFIED., .F., .F. ) 
 B_SPLINE_CURVE_WITH_KNOTS ( ( 4, 4 ),
 ( 2.005774019098183203E-15, 1.490556265852237994 ),
 .UNSPECIFIED. ) 
 CURVE ( )  GEOMETRIC_REPRESENTATION_ITEM ( )  RATIONAL_B_SPLINE_CURVE ( ( 1.000000000000000000, 0.8232662051119118418, 0.8232662051119118418, 1.000000000000000000 ) ) 
 REPRESENTATION_ITEM ( '' )  );
#11644=DIRECTION ( 'NONE',  ( 0.9961946980917465444, 0.08715574274764831264, 0.000000000000000000 ) ) ;
#11719=DIRECTION ( 'NONE',  ( 0.9961946980917463224, -0.04357787137382344855, -0.07547908730516518505 ) ) ;
#11726=DIRECTION ( 'NONE',  ( -0.08715574274765379437, 0.9961946980917459893, 0.000000000000000000 ) ) ;
#11750=CIRCLE ( 'NONE', #11458, 3.999999999999985789 ) ;
#11805=UNCERTAINTY_MEASURE_WITH_UNIT (LENGTH_MEASURE( 1.000000000000000082E-05 ), #777, 'distance_accuracy_value', 'NONE');
#11835=DIRECTION ( 'NONE',  ( 0.9961946980917464334, -0.04357787137382345549, -0.07547908730516519893 ) ) ;
#11861=CARTESIAN_POINT ( 'NONE',  ( -206.1506185320109239, 215.7475848333072861, -31.15513424541605048 ) ) ;
#11887=CARTESIAN_POINT ( 'NONE',  ( -206.3689767832464668, 123.5732568625972334, -24.35733450943962453 ) ) ;
#11958=DIRECTION ( 'NONE',  ( 0.000000000000000000, 0.000000000000000000, -1.000000000000000000 ) ) ;
#11979=CARTESIAN_POINT ( 'NONE',  ( -208.0000000000000853, 174.7326106162513497, 0.000000000000000000 ) ) ;
#12049=CLOSED_SHELL ( 'NONE', ( #11551, #9586, #12134, #1899, #9650, #14884 ) ) ;
#12062=CARTESIAN_POINT ( 'NONE',  ( -208.1243352336974510, 176.1537688404888513, 3.744334046054181186 ) ) ;
#12127=VERTEX_POINT ( 'NONE', #7912 ) ;
#12134=ADVANCED_FACE ( 'NONE', ( #1184 ), #6589, .T. ) ;
#12161=VECTOR ( 'NONE', #14699, 1000.000000000000000 ) ;
#12170=EDGE_LOOP ( 'NONE', ( #8000, #1858 ) ) ;
#12190=CARTESIAN_POINT ( 'NONE',  ( -206.6026792233873550, 173.6007525171767440, 4.555693436530018126 ) ) ;
#12201=CARTESIAN_POINT ( 'NONE',  ( -207.6775903968323576, 166.3720764825075662, 1.150672365064113079 ) ) ;
#12300=( LENGTH_UNIT ( ) NAMED_UNIT ( * ) SI_UNIT ( .MILLI., .METRE. ) );
#12478=EDGE_CURVE ( 'NONE', #12567, #10750, #10359, .T. ) ;
#12567=VERTEX_POINT ( 'NONE', #16649 ) ;
#12583=DIRECTION ( 'NONE',  ( 0.9961946980917461003, -0.04357787137382522491, -0.07547908730516825204 ) ) ;
#12602=CARTESIAN_POINT ( 'NONE',  ( -208.3486229709906752, 168.0754701982166068, -6.144114920819716552 ) ) ;
#12611=DIRECTION ( 'NONE',  ( -0.000000000000000000, 0.8660254037844432595, -0.4999999999999919509 ) ) ;
#12674=CARTESIAN_POINT ( 'NONE',  ( -208.0706889292729045, 166.1570757162849077, -1.826518625235456383 ) ) ;
#12675=( GEOMETRIC_REPRESENTATION_CONTEXT ( 3 ) GLOBAL_UNCERTAINTY_ASSIGNED_CONTEXT ( ( #11418 ) ) GLOBAL_UNIT_ASSIGNED_CONTEXT ( ( #6618, #10505, #10321 ) ) REPRESENTATION_CONTEXT ( 'NONE', 'WORKASPACE' ) );
#12708=ORIENTED_EDGE ( 'NONE', *, *, #849, .T. ) ;
#12766=CARTESIAN_POINT ( 'NONE',  ( -206.8260782938592683, 166.6501392256166127, -0.6181867824018475455 ) ) ;
#12819=DIRECTION ( 'NONE',  ( 0.9961946980917464334, -0.04357787137382450326, 0.07547908730516456055 ) ) ;
#12840=UNCERTAINTY_MEASURE_WITH_UNIT (LENGTH_MEASURE( 1.000000000000000082E-05 ), #15910, 'distance_accuracy_value', 'NONE');
#12846=ADVANCED_FACE ( 'NONE', ( #6054 ), #7551, .T. ) ;
#12853=VERTEX_POINT ( 'NONE', #13553 ) ;
#12894=LINE ( 'NONE', #15895, #5524 ) ;
#12908=ADVANCED_BREP_SHAPE_REPRESENTATION ( '', ( #11096, #11475, #5484, #3583 ), #12675 ) ;
#12961=VERTEX_POINT ( 'NONE', #2751 ) ;
#12966=CARTESIAN_POINT ( 'NONE',  ( -207.9324504923922348, 175.6261042361158786, -3.902623366482125267 ) ) ;
#12996=DIRECTION ( 'NONE',  ( 0.9961946980917464334, 0.08715574274764831264, 0.000000000000000000 ) ) ;
#13045=CARTESIAN_POINT ( 'NONE',  ( -208.1430079281944074, 172.4097984991905150, 5.932774073184737595 ) ) ;
#13080=PLANE ( 'NONE',  #14949 ) ;
#13167=EDGE_CURVE ( 'NONE', #5890, #15563, #13500, .T. ) ;
#13201=CYLINDRICAL_SURFACE ( 'NONE', #2796, 4.000000000000003553 ) ;
#13242=CARTESIAN_POINT ( 'NONE',  ( -168.0000000000000284, 178.2321571572880146, 0.000000000000000000 ) ) ;
#13268=CARTESIAN_POINT ( 'NONE',  ( -207.8780901672883772, 173.0692040606395778, -5.343448167864359277 ) ) ;
#13319=CARTESIAN_POINT ( 'NONE',  ( -207.7491074081026454, 175.3340477608625463, -3.959435662344279905 ) ) ;
#13358=PLANE ( 'NONE',  #15 ) ;
#13370=DIRECTION ( 'NONE',  ( -0.08715574274764689711, 0.9961946980917465444, 0.000000000000000000 ) ) ;
#13400=CARTESIAN_POINT ( 'NONE',  ( -208.0706889292728476, 175.9374385743225560, -3.820176503624857389 ) ) ;
#13462=CARTESIAN_POINT ( 'NONE',  ( -206.1506185320109239, 122.5792347710271741, -22.63563774299437625 ) ) ;
#13488=AXIS2_PLACEMENT_3D ( 'NONE', #11128, #8219, #4328 ) ;
#13500=CIRCLE ( 'NONE', #14618, 4.000000000000002665 ) ;
#13517=CARTESIAN_POINT ( 'NONE',  ( -207.8765633999775275, 173.0709657280817453, 5.341470372219078833 ) ) ;
#13553=CARTESIAN_POINT ( 'NONE',  ( -208.1430079281944074, 166.0913325906388422, -2.284806080016993590 ) ) ;
#13560=VERTEX_POINT ( 'NONE', #15200 ) ;
#13616=VERTEX_POINT ( 'NONE', #3595 ) ;
#13622=EDGE_CURVE ( 'NONE', #13560, #2470, #6424, .T. ) ;
#13671=CARTESIAN_POINT ( 'NONE',  ( -206.3689767832464668, 173.6103877383153531, -4.531616471133038004 ) ) ;
#13728=CARTESIAN_POINT ( 'NONE',  ( -208.3486229709906468, 168.0754701982165500, 6.144114920819691683 ) ) ;
#13733=( GEOMETRIC_REPRESENTATION_CONTEXT ( 3 ) GLOBAL_UNCERTAINTY_ASSIGNED_CONTEXT ( ( #2424 ) ) GLOBAL_UNIT_ASSIGNED_CONTEXT ( ( #9338, #2260, #6247 ) ) REPRESENTATION_CONTEXT ( 'NONE', 'WORKASPACE' ) );
#13787=EDGE_LOOP ( 'NONE', ( #5039, #9432, #16942, #16503 ) ) ;
#13820=EDGE_CURVE ( 'NONE', #12853, #6658, #5887, .T. ) ;
#13828=ORIENTED_EDGE ( 'NONE', *, *, #15816, .T. ) ;
#13831=ORIENTED_EDGE ( 'NONE', *, *, #17458, .T. ) ;
#13840=CARTESIAN_POINT ( 'NONE',  ( -207.7491074081026170, 166.3381691538542384, -1.234337273009209701 ) ) ;
#13865=DIRECTION ( 'NONE',  ( 0.9961946980917461003, -0.04357787137382522491, -0.07547908730516825204 ) ) ;
#13908=DIRECTION ( 'NONE',  ( -0.08715574274764653628, -0.4980973490458781017, 0.8627299156628190913 ) ) ;
#13923=CARTESIAN_POINT ( 'NONE',  ( -208.1430079281944074, 166.0913325906388422, -2.284806080016993590 ) ) ;
#13925=CARTESIAN_POINT ( 'NONE',  ( -208.0000000000000853, 174.7326106162513497, 53.79077198841061147 ) ) ;
#13977=PLANE ( 'NONE',  #2760 ) ;
#13991=DIRECTION ( 'NONE',  ( -0.08715574274764831264, -0.4980973490458652231, -0.8627299156628261967 ) ) ;
#14003=EDGE_CURVE ( 'NONE', #15793, #12127, #4898, .T. ) ;
#14007=CARTESIAN_POINT ( 'NONE',  ( -207.4350753193408536, 166.4757156568063294, -0.9174036676442806071 ) ) ;
#14008=CARTESIAN_POINT ( 'NONE',  ( -208.0000000000000853, 170.0678595944000620, -2.693195258168412654 ) ) ;
#14021=AXIS2_PLACEMENT_3D ( 'NONE', #13242, #11644, #859 ) ;
#14037=( BOUNDED_CURVE ( )  B_SPLINE_CURVE ( 3, ( #15257, #9590, #14994, #13671 ),
 .UNSPECIFIED., .F., .F. ) 
 B_SPLINE_CURVE_WITH_KNOTS ( ( 4, 4 ),
 ( -1.776356839400250465E-15, 1.490556265852239326 ),
 .UNSPECIFIED. ) 
 CURVE ( )  GEOMETRIC_REPRESENTATION_ITEM ( )  RATIONAL_B_SPLINE_CURVE ( ( 1.000000000000000000, 0.8232662051119106206, 0.8232662051119106206, 1.000000000000000000 ) ) 
 REPRESENTATION_ITEM ( '' )  );
#14039=ADVANCED_FACE ( 'NONE', ( #9136 ), #14543, .F. ) ;
#14049=VECTOR ( 'NONE', #10085, 1000.000000000000000 ) ;
#14051=AXIS2_PLACEMENT_3D ( 'NONE', #2747, #14702, #13370 ) ;
#14167=LINE ( 'NONE', #9004, #7861 ) ;
#14186=CARTESIAN_POINT ( 'NONE',  ( -207.2467692809710229, 166.5426260787756974, -0.7960839355505516801 ) ) ;
#14193=ORIENTED_EDGE ( 'NONE', *, *, #935, .T. ) ;
#14211=LINE ( 'NONE', #664, #3700 ) ;
#14213=CYLINDRICAL_SURFACE ( 'NONE', #1393, 2.000000000000001776 ) ;
#14231=PRESENTATION_STYLE_ASSIGNMENT (( #3350 ) ) ;
#14235=ORIENTED_EDGE ( 'NONE', *, *, #3971, .F. ) ;
#14257=DIRECTION ( 'NONE',  ( 0.9961946980917465444, -0.04357787137382451714, 0.07547908730516460218 ) ) ;
#14284=CARTESIAN_POINT ( 'NONE',  ( -208.0000000000000853, 216.6520346255402956, -29.58858125237329162 ) ) ;
#14408=CARTESIAN_POINT ( 'NONE',  ( -187.6513770290095238, 172.4976050944027008, 4.898587196589412829E-16 ) ) ;
#14463=AXIS2_PLACEMENT_3D ( 'NONE', #13925, #195, #1616 ) ;
#14473=ADVANCED_FACE ( 'NONE', ( #2589 ), #13201, .T. ) ;
#14498=PLANE ( 'NONE',  #6901 ) ;
#14516=CARTESIAN_POINT ( 'NONE',  ( -208.0000000000000853, 170.0678595944000620, -2.693195258168412654 ) ) ;
#14543=PLANE ( 'NONE',  #1368 ) ;
#14612=DIRECTION ( 'NONE',  ( 0.000000000000000000, -0.8660254037844432595, 0.4999999999999919509 ) ) ;
#14618=AXIS2_PLACEMENT_3D ( 'NONE', #15218, #3095, #13908 ) ;
#14642=CARTESIAN_POINT ( 'NONE',  ( -207.4350753193408821, 174.9908019558275498, -3.998783699268500413 ) ) ;
#14650=UNCERTAINTY_MEASURE_WITH_UNIT (LENGTH_MEASURE( 1.000000000000000082E-05 ), #12300, 'distance_accuracy_value', 'NONE');
#14679=CARTESIAN_POINT ( 'NONE',  ( -187.6513770290094669, 171.1853623553243722, -0.7576236986489900405 ) ) ;
#14690=EDGE_CURVE ( 'NONE', #12127, #5890, #4205, .T. ) ;
#14699=DIRECTION ( 'NONE',  ( 0.000000000000000000, -0.8660254037844432595, 0.4999999999999919509 ) ) ;
#14702=DIRECTION ( 'NONE',  ( 0.9961946980917465444, 0.08715574274764831264, 0.000000000000000000 ) ) ;
#14708=CARTESIAN_POINT ( 'NONE',  ( -208.1430079281944074, 176.3671987152221448, 3.647967993167786194 ) ) ;
#14727=CARTESIAN_POINT ( 'NONE',  ( -208.1430079281944074, 176.3671987152221448, 0.000000000000000000 ) ) ;
#14742=EDGE_CURVE ( 'NONE', #5523, #6530, #824, .T. ) ;
#14764=( NAMED_UNIT ( * ) PLANE_ANGLE_UNIT ( ) SI_UNIT ( $, .RADIAN. ) );
#14775=ORIENTED_EDGE ( 'NONE', *, *, #14742, .T. ) ;
#14858=PLANE ( 'NONE',  #13488 ) ;
#14871=DIRECTION ( 'NONE',  ( -1.000000000000000000, 0.000000000000000000, 0.000000000000000000 ) ) ;
#14873=( NAMED_UNIT ( * ) PLANE_ANGLE_UNIT ( ) SI_UNIT ( $, .RADIAN. ) );
#14884=ADVANCED_FACE ( 'NONE', ( #8627 ), #14213, .T. ) ;
#14892=CARTESIAN_POINT ( 'NONE',  ( -208.0000000000000853, 174.7326106162513497, 0.000000000000000000 ) ) ;
#14941=EDGE_CURVE ( 'NONE', #15663, #12567, #8651, .T. ) ;
#14949=AXIS2_PLACEMENT_3D ( 'NONE', #15908, #12996, #6616 ) ;
#14961=SURFACE_STYLE_FILL_AREA ( #16298 ) ;
#14994=CARTESIAN_POINT ( 'NONE',  ( -195.2299705378136991, 174.0696332146309544, -3.384031243670033273 ) ) ;
#15086=CARTESIAN_POINT ( 'NONE',  ( -208.1243153690002430, 172.6001711966515018, 5.795976030063606288 ) ) ;
#15092=VERTEX_POINT ( 'NONE', #15251 ) ;
#15100=CARTESIAN_POINT ( 'NONE',  ( -206.3689767832464668, 166.7044760491588988, 0.5444864983987496299 ) ) ;
#15189=CARTESIAN_POINT ( 'NONE',  ( -195.2299705378136423, 167.4686912709917408, -0.4270243643951285861 ) ) ;
#15200=CARTESIAN_POINT ( 'NONE',  ( -167.6513770290094385, 170.3104757200652273, 2.272971801780875989 ) ) ;
#15218=CARTESIAN_POINT ( 'NONE',  ( -208.0000000000000853, 170.0678595944000620, 2.693195258168412654 ) ) ;
#15247=ORIENTED_EDGE ( 'NONE', *, *, #6100, .T. ) ;
#15251=CARTESIAN_POINT ( 'NONE',  ( -187.6513770290095238, 172.4976050944027008, 4.898587196589412829E-16 ) ) ;
#15257=CARTESIAN_POINT ( 'NONE',  ( -187.6513770290094669, 171.1853623553243722, -0.7576236986489900405 ) ) ;
#15387=CARTESIAN_POINT ( 'NONE',  ( -208.1430079281944074, 172.4097984991905435, -5.932774073184737595 ) ) ;
#15396=STYLED_ITEM ( 'NONE', ( #2663 ), #11096 ) ;
#15411=CYLINDRICAL_SURFACE ( 'NONE', #6353, 3.999999999999999556 ) ;
#15440=ORIENTED_EDGE ( 'NONE', *, *, #849, .F. ) ;
#15470=FILL_AREA_STYLE ('',( #15720 ) ) ;
#15474=CARTESIAN_POINT ( 'NONE',  ( -168.0000000000000284, 168.3180863238817437, 5.723891464432140808 ) ) ;
#15503=CARTESIAN_POINT ( 'NONE',  ( -207.8765633999775275, 166.2728330025812227, -1.416566613164573774 ) ) ;
#15542=CARTESIAN_POINT ( 'NONE',  ( -206.3689767832464668, 174.5534660175772785, 3.987129972734268168 ) ) ;
#15563=VERTEX_POINT ( 'NONE', #13728 ) ;
#15663=VERTEX_POINT ( 'NONE', #9702 ) ;
#15695=CIRCLE ( 'NONE', #8068, 3.999999999999998668 ) ;
#15710=SURFACE_STYLE_USAGE ( .BOTH. , #10664 ) ;
#15720=FILL_AREA_STYLE_COLOUR ( '', #7779 ) ;
#15721=VECTOR ( 'NONE', #5430, 1000.000000000000000 ) ;
#15729=( NAMED_UNIT ( * ) SI_UNIT ( $, .STERADIAN. ) SOLID_ANGLE_UNIT ( ) );
#15745=ORIENTED_EDGE ( 'NONE', *, *, #17159, .F. ) ;
#15778=VECTOR ( 'NONE', #16289, 999.9999999999998863 ) ;
#15780=EDGE_CURVE ( 'NONE', #6530, #5523, #6664, .T. ) ;
#15793=VERTEX_POINT ( 'NONE', #10393 ) ;
#15804=PRESENTATION_STYLE_ASSIGNMENT (( #15710 ) ) ;
#15816=EDGE_CURVE ( 'NONE', #15563, #2470, #12894, .T. ) ;
#15821=EDGE_LOOP ( 'NONE', ( #4290, #8370, #17260, #8622, #323, #15980 ) ) ;
#15833=CARTESIAN_POINT ( 'NONE',  ( -207.4300157105866163, 173.3938951205217904, -4.922080471250932732 ) ) ;
#15839=( BOUNDED_CURVE ( )  B_SPLINE_CURVE ( 3, ( #2357, #7748, #4852, #14408 ),
 .UNSPECIFIED., .F., .F. ) 
 B_SPLINE_CURVE_WITH_KNOTS ( ( 4, 4 ),
 ( 4.792629041327348460, 6.283185307179586232 ),
 .UNSPECIFIED. ) 
 CURVE ( )  GEOMETRIC_REPRESENTATION_ITEM ( )  RATIONAL_B_SPLINE_CURVE ( ( 1.000000000000000000, 0.8232662051119113977, 0.8232662051119113977, 1.000000000000000000 ) ) 
 REPRESENTATION_ITEM ( '' )  );
#15869=EDGE_CURVE ( 'NONE', #7172, #6658, #15695, .T. ) ;
#15895=CARTESIAN_POINT ( 'NONE',  ( -208.3486229709906752, 168.0754701982165500, 6.144114920819689907 ) ) ;
#15908=CARTESIAN_POINT ( 'NONE',  ( -168.0000000000000284, 178.2321571572880146, 0.000000000000000000 ) ) ;
#15910=( LENGTH_UNIT ( ) NAMED_UNIT ( * ) SI_UNIT ( .MILLI., .METRE. ) );
#15917=CARTESIAN_POINT ( 'NONE',  ( -207.1416055535977705, 173.4984539563251360, -4.752130938829821183 ) ) ;
#15967=ORIENTED_EDGE ( 'NONE', *, *, #3738, .T. ) ;
#15980=ORIENTED_EDGE ( 'NONE', *, *, #10242, .T. ) ;
#16060=VERTEX_POINT ( 'NONE', #7113 ) ;
#16115=PRODUCT_DEFINITION_CONTEXT ( 'detailed design', #3142, 'design' ) ;
#16124=LINE ( 'NONE', #10707, #12161 ) ;
#16126=CARTESIAN_POINT ( 'NONE',  ( -168.0000000000000284, 168.3180863238817437, 5.723891464432140808 ) ) ;
#16151=CARTESIAN_POINT ( 'NONE',  ( -207.9328752093750836, 175.6269124087689590, 3.902437508284943846 ) ) ;
#16185=DIRECTION ( 'NONE',  ( 0.9961946980917461003, -0.04357787137382522491, -0.07547908730516825204 ) ) ;
#16195=CARTESIAN_POINT ( 'NONE',  ( -206.8291083847463767, 173.5730938514649324, -4.616715689291535973 ) ) ;
#16203=ORIENTED_EDGE ( 'NONE', *, *, #2132, .T. ) ;
#16216=SURFACE_SIDE_STYLE ('',( #14961 ) ) ;
#16219=EDGE_CURVE ( 'NONE', #16060, #13616, #7284, .T. ) ;
#16259=CARTESIAN_POINT ( 'NONE',  ( -207.4350753193408252, 173.4018121924175944, 4.916187366912743606 ) ) ;
#16287=CLOSED_SHELL ( 'NONE', ( #17059, #6888, #4896, #11168, #14039, #9752 ) ) ;
#16289=DIRECTION ( 'NONE',  ( -0.000000000000000000, -0.8660254037844363761, -0.5000000000000039968 ) ) ;
#16298=FILL_AREA_STYLE ('',( #9556 ) ) ;
#16322=EDGE_LOOP ( 'NONE', ( #9306, #11485, #5543, #4193 ) ) ;
#16330=CARTESIAN_POINT ( 'NONE',  ( -208.1430079281944074, 176.3671987152221448, -3.647967993167786194 ) ) ;
#16340=PRODUCT_CONTEXT ( 'NONE', #1332, 'mechanical' ) ;
#16367=CARTESIAN_POINT ( 'NONE',  ( -206.6025269363104826, 166.6884528440272106, 0.5648560453502019518 ) ) ;
#16503=ORIENTED_EDGE ( 'NONE', *, *, #2529, .F. ) ;
#16522=ORIENTED_EDGE ( 'NONE', *, *, #3173, .T. ) ;
#16622=ADVANCED_FACE ( 'NONE', ( #1581 ), #14858, .F. ) ;
#16649=CARTESIAN_POINT ( 'NONE',  ( -208.1430079281944074, 176.3671987152221448, -3.647967993167786194 ) ) ;
#16670=CARTESIAN_POINT ( 'NONE',  ( -208.1243153690002714, 166.1146168224391886, -2.051539466268182732 ) ) ;
#16727=DIRECTION ( 'NONE',  ( -0.08715574274764661955, -0.4980973490458647235, -0.8627299156628267518 ) ) ;
#16822=ORIENTED_EDGE ( 'NONE', *, *, #14003, .T. ) ;
#16842=COLOUR_RGB ( '', 0.31764706, 0.68627451, 0.89019608) ;
#16851=ADVANCED_FACE ( 'NONE', ( #3177 ), #13977, .T. ) ;
#16929=ORIENTED_EDGE ( 'NONE', *, *, #14690, .F. ) ;
#16942=ORIENTED_EDGE ( 'NONE', *, *, #6258, .F. ) ;
#16958=ORIENTED_EDGE ( 'NONE', *, *, #6993, .F. ) ;
#16966=CARTESIAN_POINT ( 'NONE',  ( -187.6513770290094385, 171.1853623553244006, 0.7576236986490064718 ) ) ;
#17001=LINE ( 'NONE', #3371, #14049 ) ;
#17059=ADVANCED_FACE ( 'NONE', ( #9613 ), #1302, .T. ) ;
#17071=CARTESIAN_POINT ( 'NONE',  ( -168.3486229709906183, 166.3256969276982886, -9.174811127083483342 ) ) ;
#17093=EDGE_LOOP ( 'NONE', ( #14193, #13831, #5783 ) ) ;
#17129=DIRECTION ( 'NONE',  ( -0.08715574274764661955, -0.4980973490458647235, -0.8627299156628267518 ) ) ;
#17159=EDGE_CURVE ( 'NONE', #1460, #15793, #11639, .T. ) ;
#17193=VERTEX_POINT ( 'NONE', #15542 ) ;
#17202=ORIENTED_EDGE ( 'NONE', *, *, #14003, .F. ) ;
#17238=ORIENTED_EDGE ( 'NONE', *, *, #1619, .T. ) ;
#17239=SURFACE_STYLE_FILL_AREA ( #6535 ) ;
#17249=CARTESIAN_POINT ( 'NONE',  ( -208.1243352336975079, 172.5999688864191910, -5.796121406182466629 ) ) ;
#17260=ORIENTED_EDGE ( 'NONE', *, *, #6807, .F. ) ;
#17331=CARTESIAN_POINT ( 'NONE',  ( -195.2299705378136991, 167.4686912709917124, 0.4270243643950926149 ) ) ;
#17393=CARTESIAN_POINT ( 'NONE',  ( -168.3486229709906183, 182.2169359496550101, 0.000000000000000000 ) ) ;
#17430=B_SPLINE_CURVE_WITH_KNOTS ( 'NONE', 3,
 ( #4448, #11252, #12766, #14186, #14007, #637, #13840, #15503, #1706, #12674, #16670, #13923 ),
 .UNSPECIFIED., .F., .F.,
 ( 4, 2, 2, 2, 2, 4 ),
 ( 0.000000000000000000, 0.0006954760458706877755, 0.001390952091741375551, 0.001738690114676747682, 0.002086428137612120030, 0.002781904183482844777 ),
 .UNSPECIFIED. ) ;
#17443=DIRECTION ( 'NONE',  ( 0.9961946980917463224, -0.04357787137382344855, -0.07547908730516518505 ) ) ;
#17458=EDGE_CURVE ( 'NONE', #15092, #17193, #4417, .T. ) ;
#17471=CARTESIAN_POINT ( 'NONE',  ( -208.0711340499744324, 175.9387398585090523, 3.819775182827789717 ) ) ;
ENDSEC;
END-ISO-10303-21;
